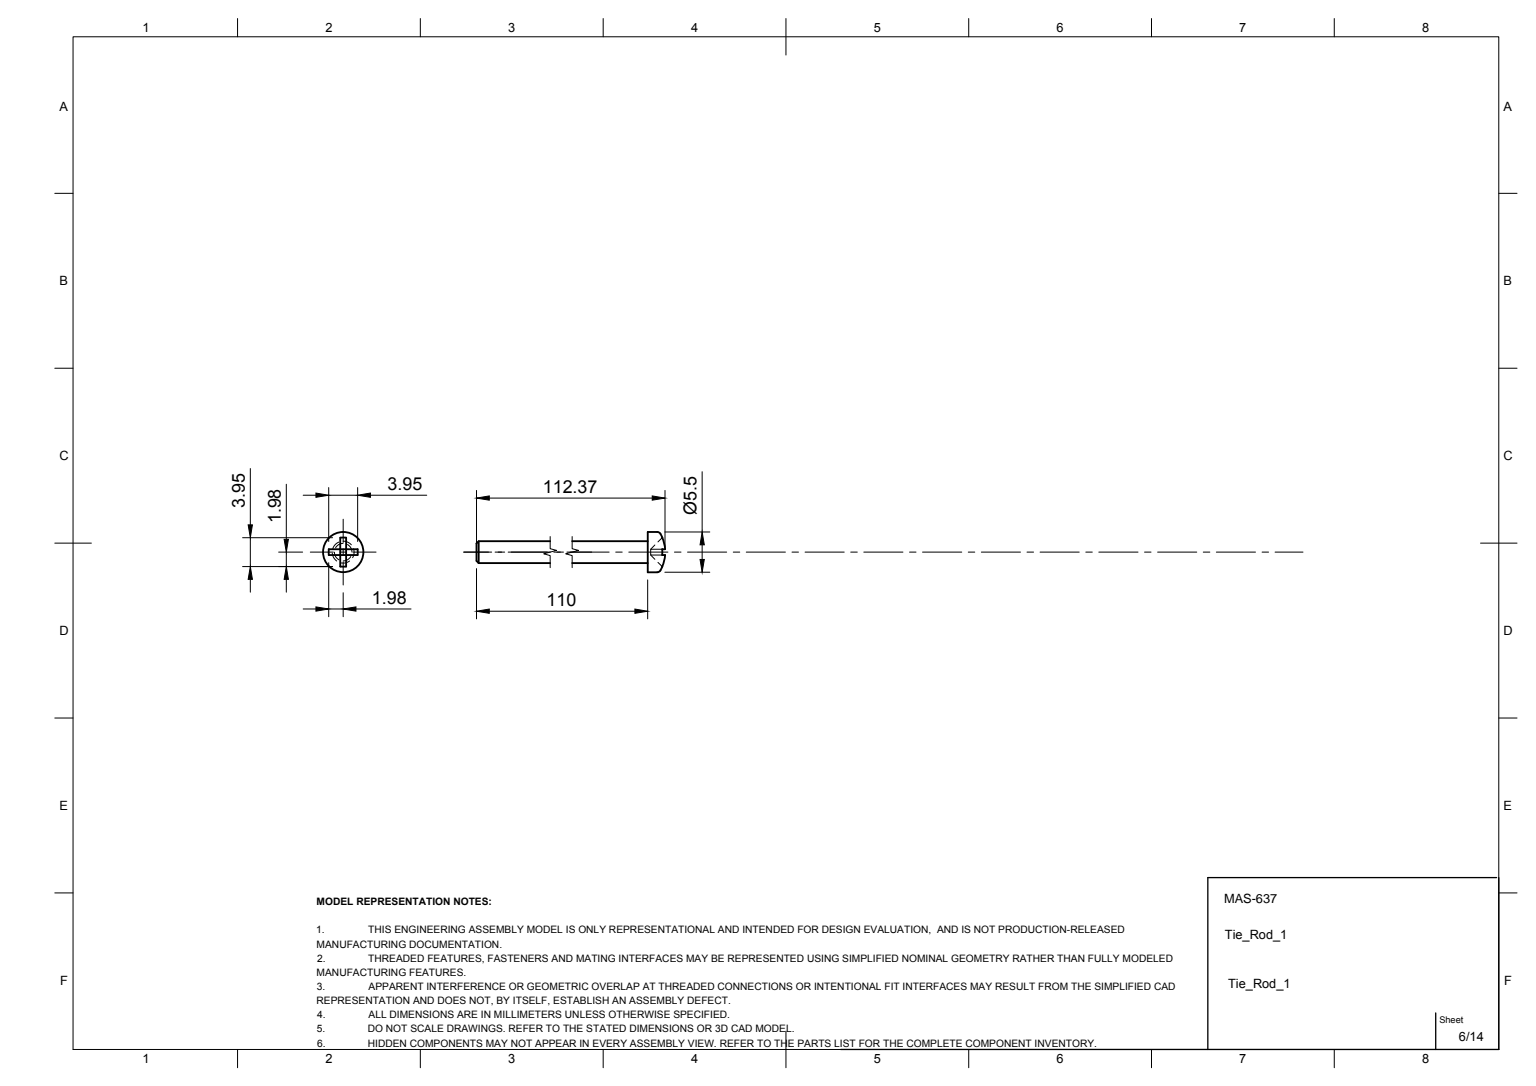
ISO-10303-21;
HEADER;
FILE_DESCRIPTION((''),'2;1');
FILE_NAME('Tie_Rod_1.step','2026-10-09T10:11:57-07:00',(''),(''),'','','');
FILE_SCHEMA (('AUTOMOTIVE_DESIGN { 1 0 10303 214 3 1 1 }'));
ENDSEC;
DATA;
#10=MECHANICAL_DESIGN_GEOMETRIC_PRESENTATION_REPRESENTATION('',(#126),#13510);
#71=SPHERICAL_SURFACE('',#8066,5.) ;
#96=SHAPE_REPRESENTATION_RELATIONSHIP('SRR','None',#13566,#111) ;
#111=ADVANCED_BREP_SHAPE_REPRESENTATION('',(#158),#13498) ;
#126=STYLED_ITEM('',(#13650),#158) ;
#158=MANIFOLD_SOLID_BREP('Body1',#7375) ;
#240=FACE_BOUND('',#1372,.T.) ;
#352=PLANE('',#8051) ;
#353=PLANE('',#8052) ;
#354=PLANE('',#8053) ;
#355=PLANE('',#8055) ;
#356=PLANE('',#8057) ;
#357=PLANE('',#8060) ;
#358=PLANE('',#8062) ;
#359=PLANE('',#8064) ;
#360=PLANE('',#8074) ;
#361=PLANE('',#8075) ;
#362=PLANE('',#8076) ;
#363=PLANE('',#8077) ;
#364=PLANE('',#8078) ;
#365=PLANE('',#8079) ;
#366=PLANE('',#8080) ;
#498=TOROIDAL_SURFACE('',#8040,2.25,0.5) ;
#632=CYLINDRICAL_SURFACE('',#8044,2.75) ;
#633=CYLINDRICAL_SURFACE('',#8046,1.5) ;
#866=FACE_OUTER_BOUND('',#1367,.T.) ;
#867=FACE_OUTER_BOUND('',#1368,.T.) ;
#868=FACE_OUTER_BOUND('',#1369,.T.) ;
#869=FACE_OUTER_BOUND('',#1370,.T.) ;
#870=FACE_OUTER_BOUND('',#1371,.T.) ;
#871=FACE_OUTER_BOUND('',#1373,.T.) ;
#872=FACE_OUTER_BOUND('',#1374,.T.) ;
#873=FACE_OUTER_BOUND('',#1375,.T.) ;
#874=FACE_OUTER_BOUND('',#1376,.T.) ;
#875=FACE_OUTER_BOUND('',#1377,.T.) ;
#876=FACE_OUTER_BOUND('',#1378,.T.) ;
#877=FACE_OUTER_BOUND('',#1379,.T.) ;
#878=FACE_OUTER_BOUND('',#1380,.T.) ;
#879=FACE_OUTER_BOUND('',#1381,.T.) ;
#880=FACE_OUTER_BOUND('',#1382,.T.) ;
#881=FACE_OUTER_BOUND('',#1383,.T.) ;
#882=FACE_OUTER_BOUND('',#1384,.T.) ;
#883=FACE_OUTER_BOUND('',#1385,.T.) ;
#884=FACE_OUTER_BOUND('',#1386,.T.) ;
#885=FACE_OUTER_BOUND('',#1387,.T.) ;
#1367=EDGE_LOOP('',(#5906,#5907,#5908,#5909)) ;
#1368=EDGE_LOOP('',(#5910,#5911,#5912,#5913)) ;
#1369=EDGE_LOOP('',(#5914,#5915,#5916,#5917)) ;
#1370=EDGE_LOOP('',(#5918,#5919,#5920,#5921)) ;
#1371=EDGE_LOOP('',(#5922)) ;
#1372=EDGE_LOOP('',(#5923)) ;
#1373=EDGE_LOOP('',(#5924)) ;
#1374=EDGE_LOOP('',(#5925,#5926,#5927,#5928)) ;
#1375=EDGE_LOOP('',(#5929,#5930,#5931,#5932)) ;
#1376=EDGE_LOOP('',(#5933,#5934,#5935,#5936)) ;
#1377=EDGE_LOOP('',(#5937,#5938,#5939)) ;
#1378=EDGE_LOOP('',(#5940,#5941,#5942)) ;
#1379=EDGE_LOOP('',(#5943,#5944,#5945)) ;
#1380=EDGE_LOOP('',(#5946,#5947,#5948,#5949,#5950,#5951,#5952,#5953,#5954,
#5955,#5956,#5957,#5958,#5959,#5960,#5961)) ;
#1381=EDGE_LOOP('',(#5962,#5963,#5964)) ;
#1382=EDGE_LOOP('',(#5965,#5966,#5967,#5968)) ;
#1383=EDGE_LOOP('',(#5969,#5970,#5971)) ;
#1384=EDGE_LOOP('',(#5972,#5973,#5974)) ;
#1385=EDGE_LOOP('',(#5975,#5976,#5977,#5978)) ;
#1386=EDGE_LOOP('',(#5979,#5980,#5981)) ;
#1387=EDGE_LOOP('',(#5982,#5983,#5984,#5985)) ;
#1906=LINE('',#12420,#2400) ;
#1907=LINE('',#12425,#2401) ;
#1908=LINE('',#12429,#2402) ;
#1909=LINE('',#12436,#2403) ;
#1910=LINE('',#12438,#2404) ;
#1911=LINE('',#12440,#2405) ;
#1912=LINE('',#12447,#2406) ;
#1913=LINE('',#12449,#2407) ;
#1914=LINE('',#12450,#2408) ;
#1915=LINE('',#12453,#2409) ;
#1916=LINE('',#12459,#2410) ;
#1917=LINE('',#12464,#2411) ;
#1918=LINE('',#12468,#2412) ;
#1919=LINE('',#12482,#2413) ;
#1920=LINE('',#12484,#2414) ;
#1921=LINE('',#12485,#2415) ;
#1922=LINE('',#12488,#2416) ;
#1923=LINE('',#12490,#2417) ;
#1924=LINE('',#12491,#2418) ;
#2400=VECTOR('',#9776,2.75) ;
#2401=VECTOR('',#9781,1.5) ;
#2402=VECTOR('',#9786,1.2) ;
#2403=VECTOR('',#9795,1.00000000000064) ;
#2404=VECTOR('',#9796,1.) ;
#2405=VECTOR('',#9797,1.00000000000064) ;
#2406=VECTOR('',#9804,1.00000000000064) ;
#2407=VECTOR('',#9805,1.) ;
#2408=VECTOR('',#9806,1.00000000000064) ;
#2409=VECTOR('',#9809,1.) ;
#2410=VECTOR('',#9816,1.) ;
#2411=VECTOR('',#9823,1.) ;
#2412=VECTOR('',#9828,1.) ;
#2413=VECTOR('',#9847,1.00000000000064) ;
#2414=VECTOR('',#9850,1.00000000000064) ;
#2415=VECTOR('',#9851,1.) ;
#2416=VECTOR('',#9856,1.00000000000064) ;
#2417=VECTOR('',#9859,1.) ;
#2418=VECTOR('',#9860,1.00000000000064) ;
#2898=CIRCLE('',#8041,2.75) ;
#2899=CIRCLE('',#8042,0.5) ;
#2900=CIRCLE('',#8043,2.5) ;
#2901=CIRCLE('',#8045,2.75) ;
#2902=CIRCLE('',#8047,1.5) ;
#2903=CIRCLE('',#8048,1.5) ;
#2904=CIRCLE('',#8050,1.2) ;
#2905=CIRCLE('',#8054,4.64997588898226) ;
#2906=CIRCLE('',#8056,4.64997588898056) ;
#2907=CIRCLE('',#8058,4.98397431775085) ;
#2908=CIRCLE('',#8059,4.98397431775085) ;
#2909=CIRCLE('',#8061,4.9839617983173) ;
#2910=CIRCLE('',#8063,4.98396179831711) ;
#2911=CIRCLE('',#8065,4.98397431775085) ;
#2912=CIRCLE('',#8067,5.) ;
#2913=CIRCLE('',#8068,4.98397431775085) ;
#2914=CIRCLE('',#8069,4.64973117502507) ;
#2915=CIRCLE('',#8070,4.98397431775085) ;
#2916=CIRCLE('',#8071,4.98397431775085) ;
#2917=CIRCLE('',#8072,4.64973117502507) ;
#2918=CIRCLE('',#8073,4.98397431775085) ;
#3496=VERTEX_POINT('',#12412) ;
#3497=VERTEX_POINT('',#12414) ;
#3498=VERTEX_POINT('',#12418) ;
#3499=VERTEX_POINT('',#12422) ;
#3500=VERTEX_POINT('',#12424) ;
#3501=VERTEX_POINT('',#12428) ;
#3502=VERTEX_POINT('',#12434) ;
#3503=VERTEX_POINT('',#12435) ;
#3504=VERTEX_POINT('',#12437) ;
#3505=VERTEX_POINT('',#12439) ;
#3506=VERTEX_POINT('',#12443) ;
#3507=VERTEX_POINT('',#12444) ;
#3508=VERTEX_POINT('',#12446) ;
#3509=VERTEX_POINT('',#12448) ;
#3510=VERTEX_POINT('',#12452) ;
#3511=VERTEX_POINT('',#12454) ;
#3512=VERTEX_POINT('',#12458) ;
#3513=VERTEX_POINT('',#12462) ;
#3514=VERTEX_POINT('',#12466) ;
#3515=VERTEX_POINT('',#12471) ;
#3516=VERTEX_POINT('',#12473) ;
#3517=VERTEX_POINT('',#12476) ;
#3518=VERTEX_POINT('',#12478) ;
#4340=EDGE_CURVE('',#3496,#3496,#2898,.T.) ;
#4341=EDGE_CURVE('',#3496,#3497,#2899,.T.) ;
#4342=EDGE_CURVE('',#3497,#3497,#2900,.T.) ;
#4343=EDGE_CURVE('',#3498,#3498,#2901,.T.) ;
#4344=EDGE_CURVE('',#3498,#3496,#1906,.T.) ;
#4345=EDGE_CURVE('',#3499,#3499,#2902,.T.) ;
#4346=EDGE_CURVE('',#3499,#3500,#1907,.T.) ;
#4347=EDGE_CURVE('',#3500,#3500,#2903,.T.) ;
#4348=EDGE_CURVE('',#3499,#3501,#1908,.T.) ;
#4349=EDGE_CURVE('',#3501,#3501,#2904,.F.) ;
#4350=EDGE_CURVE('',#3502,#3503,#1909,.T.) ;
#4351=EDGE_CURVE('',#3502,#3504,#1910,.F.) ;
#4352=EDGE_CURVE('',#3504,#3505,#1911,.T.) ;
#4353=EDGE_CURVE('',#3505,#3503,#2905,.T.) ;
#4354=EDGE_CURVE('',#3506,#3507,#2906,.T.) ;
#4355=EDGE_CURVE('',#3506,#3508,#1912,.F.) ;
#4356=EDGE_CURVE('',#3509,#3508,#1913,.F.) ;
#4357=EDGE_CURVE('',#3507,#3509,#1914,.F.) ;
#4358=EDGE_CURVE('',#3504,#3510,#1915,.T.) ;
#4359=EDGE_CURVE('',#3511,#3510,#2907,.F.) ;
#4360=EDGE_CURVE('',#3505,#3511,#2908,.F.) ;
#4361=EDGE_CURVE('',#3508,#3512,#1916,.T.) ;
#4362=EDGE_CURVE('',#3512,#3506,#2909,.T.) ;
#4363=EDGE_CURVE('',#3513,#3503,#2910,.T.) ;
#4364=EDGE_CURVE('',#3502,#3513,#1917,.T.) ;
#4365=EDGE_CURVE('',#3507,#3514,#2911,.F.) ;
#4366=EDGE_CURVE('',#3509,#3514,#1918,.T.) ;
#4367=EDGE_CURVE('',#3497,#3511,#2912,.T.) ;
#4368=EDGE_CURVE('',#3515,#3510,#2913,.T.) ;
#4369=EDGE_CURVE('',#3516,#3515,#2914,.T.) ;
#4370=EDGE_CURVE('',#3516,#3512,#2915,.T.) ;
#4371=EDGE_CURVE('',#3517,#3514,#2916,.T.) ;
#4372=EDGE_CURVE('',#3517,#3518,#2917,.T.) ;
#4373=EDGE_CURVE('',#3518,#3513,#2918,.T.) ;
#4374=EDGE_CURVE('',#3518,#3502,#1919,.F.) ;
#4375=EDGE_CURVE('',#3517,#3509,#1920,.F.) ;
#4376=EDGE_CURVE('',#3509,#3502,#1921,.T.) ;
#4377=EDGE_CURVE('',#3504,#3515,#1922,.T.) ;
#4378=EDGE_CURVE('',#3508,#3504,#1923,.T.) ;
#4379=EDGE_CURVE('',#3508,#3516,#1924,.T.) ;
#5906=ORIENTED_EDGE('',*,*,#4340,.F.) ;
#5907=ORIENTED_EDGE('',*,*,#4341,.T.) ;
#5908=ORIENTED_EDGE('',*,*,#4342,.T.) ;
#5909=ORIENTED_EDGE('',*,*,#4341,.F.) ;
#5910=ORIENTED_EDGE('',*,*,#4343,.F.) ;
#5911=ORIENTED_EDGE('',*,*,#4344,.T.) ;
#5912=ORIENTED_EDGE('',*,*,#4340,.T.) ;
#5913=ORIENTED_EDGE('',*,*,#4344,.F.) ;
#5914=ORIENTED_EDGE('',*,*,#4345,.F.) ;
#5915=ORIENTED_EDGE('',*,*,#4346,.T.) ;
#5916=ORIENTED_EDGE('',*,*,#4347,.T.) ;
#5917=ORIENTED_EDGE('',*,*,#4346,.F.) ;
#5918=ORIENTED_EDGE('',*,*,#4345,.T.) ;
#5919=ORIENTED_EDGE('',*,*,#4348,.T.) ;
#5920=ORIENTED_EDGE('',*,*,#4349,.F.) ;
#5921=ORIENTED_EDGE('',*,*,#4348,.F.) ;
#5922=ORIENTED_EDGE('',*,*,#4343,.T.) ;
#5923=ORIENTED_EDGE('',*,*,#4347,.F.) ;
#5924=ORIENTED_EDGE('',*,*,#4349,.T.) ;
#5925=ORIENTED_EDGE('',*,*,#4350,.F.) ;
#5926=ORIENTED_EDGE('',*,*,#4351,.T.) ;
#5927=ORIENTED_EDGE('',*,*,#4352,.T.) ;
#5928=ORIENTED_EDGE('',*,*,#4353,.T.) ;
#5929=ORIENTED_EDGE('',*,*,#4354,.F.) ;
#5930=ORIENTED_EDGE('',*,*,#4355,.T.) ;
#5931=ORIENTED_EDGE('',*,*,#4356,.F.) ;
#5932=ORIENTED_EDGE('',*,*,#4357,.F.) ;
#5933=ORIENTED_EDGE('',*,*,#4358,.T.) ;
#5934=ORIENTED_EDGE('',*,*,#4359,.F.) ;
#5935=ORIENTED_EDGE('',*,*,#4360,.F.) ;
#5936=ORIENTED_EDGE('',*,*,#4352,.F.) ;
#5937=ORIENTED_EDGE('',*,*,#4361,.F.) ;
#5938=ORIENTED_EDGE('',*,*,#4355,.F.) ;
#5939=ORIENTED_EDGE('',*,*,#4362,.F.) ;
#5940=ORIENTED_EDGE('',*,*,#4350,.T.) ;
#5941=ORIENTED_EDGE('',*,*,#4363,.F.) ;
#5942=ORIENTED_EDGE('',*,*,#4364,.F.) ;
#5943=ORIENTED_EDGE('',*,*,#4365,.F.) ;
#5944=ORIENTED_EDGE('',*,*,#4357,.T.) ;
#5945=ORIENTED_EDGE('',*,*,#4366,.T.) ;
#5946=ORIENTED_EDGE('',*,*,#4342,.F.) ;
#5947=ORIENTED_EDGE('',*,*,#4367,.T.) ;
#5948=ORIENTED_EDGE('',*,*,#4359,.T.) ;
#5949=ORIENTED_EDGE('',*,*,#4368,.F.) ;
#5950=ORIENTED_EDGE('',*,*,#4369,.F.) ;
#5951=ORIENTED_EDGE('',*,*,#4370,.T.) ;
#5952=ORIENTED_EDGE('',*,*,#4362,.T.) ;
#5953=ORIENTED_EDGE('',*,*,#4354,.T.) ;
#5954=ORIENTED_EDGE('',*,*,#4365,.T.) ;
#5955=ORIENTED_EDGE('',*,*,#4371,.F.) ;
#5956=ORIENTED_EDGE('',*,*,#4372,.T.) ;
#5957=ORIENTED_EDGE('',*,*,#4373,.T.) ;
#5958=ORIENTED_EDGE('',*,*,#4363,.T.) ;
#5959=ORIENTED_EDGE('',*,*,#4353,.F.) ;
#5960=ORIENTED_EDGE('',*,*,#4360,.T.) ;
#5961=ORIENTED_EDGE('',*,*,#4367,.F.) ;
#5962=ORIENTED_EDGE('',*,*,#4374,.T.) ;
#5963=ORIENTED_EDGE('',*,*,#4364,.T.) ;
#5964=ORIENTED_EDGE('',*,*,#4373,.F.) ;
#5965=ORIENTED_EDGE('',*,*,#4374,.F.) ;
#5966=ORIENTED_EDGE('',*,*,#4372,.F.) ;
#5967=ORIENTED_EDGE('',*,*,#4375,.T.) ;
#5968=ORIENTED_EDGE('',*,*,#4376,.T.) ;
#5969=ORIENTED_EDGE('',*,*,#4371,.T.) ;
#5970=ORIENTED_EDGE('',*,*,#4366,.F.) ;
#5971=ORIENTED_EDGE('',*,*,#4375,.F.) ;
#5972=ORIENTED_EDGE('',*,*,#4377,.T.) ;
#5973=ORIENTED_EDGE('',*,*,#4368,.T.) ;
#5974=ORIENTED_EDGE('',*,*,#4358,.F.) ;
#5975=ORIENTED_EDGE('',*,*,#4377,.F.) ;
#5976=ORIENTED_EDGE('',*,*,#4378,.F.) ;
#5977=ORIENTED_EDGE('',*,*,#4379,.T.) ;
#5978=ORIENTED_EDGE('',*,*,#4369,.T.) ;
#5979=ORIENTED_EDGE('',*,*,#4361,.T.) ;
#5980=ORIENTED_EDGE('',*,*,#4370,.F.) ;
#5981=ORIENTED_EDGE('',*,*,#4379,.F.) ;
#5982=ORIENTED_EDGE('',*,*,#4378,.T.) ;
#5983=ORIENTED_EDGE('',*,*,#4351,.F.) ;
#5984=ORIENTED_EDGE('',*,*,#4376,.F.) ;
#5985=ORIENTED_EDGE('',*,*,#4356,.T.) ;
#6885=CONICAL_SURFACE('',#8049,1.2,0.785398163397) ;
#7116=ADVANCED_FACE('',(#866),#498,.T.) ;
#7117=ADVANCED_FACE('',(#867),#632,.T.) ;
#7118=ADVANCED_FACE('',(#868),#633,.T.) ;
#7119=ADVANCED_FACE('',(#869),#6885,.T.) ;
#7120=ADVANCED_FACE('',(#870,#240),#352,.T.) ;
#7121=ADVANCED_FACE('',(#871),#353,.T.) ;
#7122=ADVANCED_FACE('',(#872),#354,.T.) ;
#7123=ADVANCED_FACE('',(#873),#355,.F.) ;
#7124=ADVANCED_FACE('',(#874),#356,.F.) ;
#7125=ADVANCED_FACE('',(#875),#357,.F.) ;
#7126=ADVANCED_FACE('',(#876),#358,.T.) ;
#7127=ADVANCED_FACE('',(#877),#359,.T.) ;
#7128=ADVANCED_FACE('',(#878),#71,.T.) ;
#7129=ADVANCED_FACE('',(#879),#360,.T.) ;
#7130=ADVANCED_FACE('',(#880),#361,.F.) ;
#7131=ADVANCED_FACE('',(#881),#362,.F.) ;
#7132=ADVANCED_FACE('',(#882),#363,.T.) ;
#7133=ADVANCED_FACE('',(#883),#364,.T.) ;
#7134=ADVANCED_FACE('',(#884),#365,.F.) ;
#7135=ADVANCED_FACE('',(#885),#366,.F.) ;
#7375=CLOSED_SHELL('',(#7116,#7117,#7118,#7119,#7120,#7121,#7122,#7123,
#7124,#7125,#7126,#7127,#7128,#7129,#7130,#7131,#7132,#7133,#7134,#7135)) ;
#8039=AXIS2_PLACEMENT_3D('',#12410,#9762,#9763) ;
#8040=AXIS2_PLACEMENT_3D('',#12411,#9764,#9765) ;
#8041=AXIS2_PLACEMENT_3D('',#12413,#9766,#9767) ;
#8042=AXIS2_PLACEMENT_3D('',#12415,#9768,#9769) ;
#8043=AXIS2_PLACEMENT_3D('',#12416,#9770,#9771) ;
#8044=AXIS2_PLACEMENT_3D('',#12417,#9772,#9773) ;
#8045=AXIS2_PLACEMENT_3D('',#12419,#9774,#9775) ;
#8046=AXIS2_PLACEMENT_3D('',#12421,#9777,#9778) ;
#8047=AXIS2_PLACEMENT_3D('',#12423,#9779,#9780) ;
#8048=AXIS2_PLACEMENT_3D('',#12426,#9782,#9783) ;
#8049=AXIS2_PLACEMENT_3D('',#12427,#9784,#9785) ;
#8050=AXIS2_PLACEMENT_3D('',#12430,#9787,#9788) ;
#8051=AXIS2_PLACEMENT_3D('',#12431,#9789,#9790) ;
#8052=AXIS2_PLACEMENT_3D('',#12432,#9791,#9792) ;
#8053=AXIS2_PLACEMENT_3D('',#12433,#9793,#9794) ;
#8054=AXIS2_PLACEMENT_3D('',#12441,#9798,#9799) ;
#8055=AXIS2_PLACEMENT_3D('',#12442,#9800,#9801) ;
#8056=AXIS2_PLACEMENT_3D('',#12445,#9802,#9803) ;
#8057=AXIS2_PLACEMENT_3D('',#12451,#9807,#9808) ;
#8058=AXIS2_PLACEMENT_3D('',#12455,#9810,#9811) ;
#8059=AXIS2_PLACEMENT_3D('',#12456,#9812,#9813) ;
#8060=AXIS2_PLACEMENT_3D('',#12457,#9814,#9815) ;
#8061=AXIS2_PLACEMENT_3D('',#12460,#9817,#9818) ;
#8062=AXIS2_PLACEMENT_3D('',#12461,#9819,#9820) ;
#8063=AXIS2_PLACEMENT_3D('',#12463,#9821,#9822) ;
#8064=AXIS2_PLACEMENT_3D('',#12465,#9824,#9825) ;
#8065=AXIS2_PLACEMENT_3D('',#12467,#9826,#9827) ;
#8066=AXIS2_PLACEMENT_3D('',#12469,#9829,#9830) ;
#8067=AXIS2_PLACEMENT_3D('',#12470,#9831,#9832) ;
#8068=AXIS2_PLACEMENT_3D('',#12472,#9833,#9834) ;
#8069=AXIS2_PLACEMENT_3D('',#12474,#9835,#9836) ;
#8070=AXIS2_PLACEMENT_3D('',#12475,#9837,#9838) ;
#8071=AXIS2_PLACEMENT_3D('',#12477,#9839,#9840) ;
#8072=AXIS2_PLACEMENT_3D('',#12479,#9841,#9842) ;
#8073=AXIS2_PLACEMENT_3D('',#12480,#9843,#9844) ;
#8074=AXIS2_PLACEMENT_3D('',#12481,#9845,#9846) ;
#8075=AXIS2_PLACEMENT_3D('',#12483,#9848,#9849) ;
#8076=AXIS2_PLACEMENT_3D('',#12486,#9852,#9853) ;
#8077=AXIS2_PLACEMENT_3D('',#12487,#9854,#9855) ;
#8078=AXIS2_PLACEMENT_3D('',#12489,#9857,#9858) ;
#8079=AXIS2_PLACEMENT_3D('',#12492,#9861,#9862) ;
#8080=AXIS2_PLACEMENT_3D('',#12493,#9863,#9864) ;
#9762=DIRECTION('axis',(0.,0.,1.)) ;
#9763=DIRECTION('refdir',(1.,0.,0.)) ;
#9764=DIRECTION('center_axis',(0.,0.,1.)) ;
#9765=DIRECTION('ref_axis',(-0.479425538604204,0.877582561890372,0.)) ;
#9766=DIRECTION('center_axis',(0.,0.,1.)) ;
#9767=DIRECTION('ref_axis',(-1.,0.,0.)) ;
#9768=DIRECTION('center_axis',(0.877582561890372,0.479425538604204,0.)) ;
#9769=DIRECTION('ref_axis',(0.479425538604204,-0.877582561890372,0.)) ;
#9770=DIRECTION('center_axis',(0.,0.,1.)) ;
#9771=DIRECTION('ref_axis',(-1.,0.,0.)) ;
#9772=DIRECTION('center_axis',(0.,0.,1.)) ;
#9773=DIRECTION('ref_axis',(-0.479425538604204,0.877582561890372,0.)) ;
#9774=DIRECTION('center_axis',(0.,0.,1.)) ;
#9775=DIRECTION('ref_axis',(-1.,0.,0.)) ;
#9776=DIRECTION('',(0.,0.,-1.)) ;
#9777=DIRECTION('center_axis',(0.,0.,1.)) ;
#9778=DIRECTION('ref_axis',(-0.479425538604204,0.877582561890372,0.)) ;
#9779=DIRECTION('center_axis',(0.,0.,1.)) ;
#9780=DIRECTION('ref_axis',(-1.,0.,0.)) ;
#9781=DIRECTION('',(0.,0.,-1.)) ;
#9782=DIRECTION('center_axis',(0.,0.,1.)) ;
#9783=DIRECTION('ref_axis',(-1.,0.,0.)) ;
#9784=DIRECTION('center_axis',(0.,0.,-1.)) ;
#9785=DIRECTION('ref_axis',(-0.479425538604203,0.877582561890373,0.)) ;
#9786=DIRECTION('',(-0.339005049420893,0.620544580563467,0.707106781186865)) ;
#9787=DIRECTION('center_axis',(0.,0.,-1.)) ;
#9788=DIRECTION('ref_axis',(1.,0.,0.)) ;
#9789=DIRECTION('center_axis',(0.,0.,1.)) ;
#9790=DIRECTION('ref_axis',(1.,0.,0.)) ;
#9791=DIRECTION('center_axis',(0.,0.,1.)) ;
#9792=DIRECTION('ref_axis',(1.,0.,0.)) ;
#9793=DIRECTION('center_axis',(0.,0.707106781186548,-0.707106781186548)) ;
#9794=DIRECTION('ref_axis',(0.,-0.707106781186548,-0.707106781186548)) ;
#9795=DIRECTION('',(0.,-0.707106781186548,-0.707106781186548)) ;
#9796=DIRECTION('',(-1.,0.,0.)) ;
#9797=DIRECTION('',(0.,-0.707106781186548,-0.707106781186548)) ;
#9798=DIRECTION('center_axis',(0.,0.70710678018955,-0.707106782183545)) ;
#9799=DIRECTION('ref_axis',(-0.0860219514143675,-0.704485708397953,-0.70448570641135)) ;
#9800=DIRECTION('center_axis',(0.,0.707106781186548,0.707106781186548)) ;
#9801=DIRECTION('ref_axis',(0.,0.707106781186548,-0.707106781186548)) ;
#9802=DIRECTION('center_axis',(0.,0.707106780189292,0.707106782183803)) ;
#9803=DIRECTION('ref_axis',(-0.0860219514143926,0.704485708398209,-0.704485706411091)) ;
#9804=DIRECTION('',(0.,0.707106781186548,-0.707106781186548)) ;
#9805=DIRECTION('',(-1.,0.,0.)) ;
#9806=DIRECTION('',(0.,0.707106781186548,-0.707106781186548)) ;
#9807=DIRECTION('center_axis',(1.,0.,0.)) ;
#9808=DIRECTION('ref_axis',(0.,1.,0.)) ;
#9809=DIRECTION('',(0.,0.,-1.)) ;
#9810=DIRECTION('center_axis',(-1.,0.,0.)) ;
#9811=DIRECTION('ref_axis',(0.,0.,1.)) ;
#9812=DIRECTION('center_axis',(-1.,0.,0.)) ;
#9813=DIRECTION('ref_axis',(0.,0.,1.)) ;
#9814=DIRECTION('center_axis',(1.,0.,0.)) ;
#9815=DIRECTION('ref_axis',(0.,1.,0.)) ;
#9816=DIRECTION('',(0.,0.,-1.)) ;
#9817=DIRECTION('center_axis',(1.,0.,0.)) ;
#9818=DIRECTION('ref_axis',(0.,0.396404687454843,-0.918075881266809)) ;
#9819=DIRECTION('center_axis',(1.,0.,0.)) ;
#9820=DIRECTION('ref_axis',(0.,1.,0.)) ;
#9821=DIRECTION('center_axis',(-1.,0.,0.)) ;
#9822=DIRECTION('ref_axis',(0.,-0.396404687454847,-0.918075881266807)) ;
#9823=DIRECTION('',(0.,0.,-1.)) ;
#9824=DIRECTION('center_axis',(1.,0.,0.)) ;
#9825=DIRECTION('ref_axis',(0.,1.,0.)) ;
#9826=DIRECTION('center_axis',(1.,0.,0.)) ;
#9827=DIRECTION('ref_axis',(0.,0.,1.)) ;
#9828=DIRECTION('',(0.,0.,-1.)) ;
#9829=DIRECTION('center_axis',(-8.80690426921701E-17,0.,1.)) ;
#9830=DIRECTION('ref_axis',(-0.479425538604204,0.877582561890372,0.)) ;
#9831=DIRECTION('center_axis',(0.877582561890372,0.479425538604204,5.15252374060181E-17)) ;
#9832=DIRECTION('ref_axis',(0.479425538604204,-0.877582561890372,0.)) ;
#9833=DIRECTION('center_axis',(6.12323399574E-17,1.,0.)) ;
#9834=DIRECTION('ref_axis',(0.,0.,-1.)) ;
#9835=DIRECTION('center_axis',(-0.707106781186548,4.32978028117723E-17,
-0.707106781186548)) ;
#9836=DIRECTION('ref_axis',(2.73536852476314E-32,-1.,-6.12323399573643E-17)) ;
#9837=DIRECTION('center_axis',(6.12323399574E-17,1.,0.)) ;
#9838=DIRECTION('ref_axis',(0.,0.,-1.)) ;
#9839=DIRECTION('center_axis',(-6.12323399574E-17,-1.,0.)) ;
#9840=DIRECTION('ref_axis',(0.,0.,-1.)) ;
#9841=DIRECTION('center_axis',(-0.707106781186548,4.32978028117723E-17,
0.707106781186548)) ;
#9842=DIRECTION('ref_axis',(-2.73536852476314E-32,1.,-6.12323399573643E-17)) ;
#9843=DIRECTION('center_axis',(-6.12323399574E-17,-1.,0.)) ;
#9844=DIRECTION('ref_axis',(0.,0.,-1.)) ;
#9845=DIRECTION('center_axis',(6.12323399574E-17,1.,0.)) ;
#9846=DIRECTION('ref_axis',(-1.,6.12323399574E-17,0.)) ;
#9847=DIRECTION('',(-0.707106781186548,0.,-0.707106781186548)) ;
#9848=DIRECTION('center_axis',(-0.707106781186548,4.32978028117723E-17,
0.707106781186548)) ;
#9849=DIRECTION('ref_axis',(-0.707106781186548,4.32978028117723E-17,-0.707106781186548)) ;
#9850=DIRECTION('',(-0.707106781186548,0.,-0.707106781186548)) ;
#9851=DIRECTION('',(0.,-1.,0.)) ;
#9852=DIRECTION('center_axis',(6.12323399574E-17,1.,0.)) ;
#9853=DIRECTION('ref_axis',(-1.,6.12323399574E-17,0.)) ;
#9854=DIRECTION('center_axis',(6.12323399574E-17,1.,0.)) ;
#9855=DIRECTION('ref_axis',(-1.,6.12323399574E-17,0.)) ;
#9856=DIRECTION('',(0.707106781186548,0.,-0.707106781186548)) ;
#9857=DIRECTION('center_axis',(-0.707106781186548,4.32978028117723E-17,
-0.707106781186548)) ;
#9858=DIRECTION('ref_axis',(0.707106781186548,-4.32978028117723E-17,-0.707106781186548)) ;
#9859=DIRECTION('',(0.,-1.,0.)) ;
#9860=DIRECTION('',(0.707106781186548,0.,-0.707106781186548)) ;
#9861=DIRECTION('center_axis',(6.12323399574E-17,1.,0.)) ;
#9862=DIRECTION('ref_axis',(-1.,6.12323399574E-17,0.)) ;
#9863=DIRECTION('center_axis',(0.,0.,1.)) ;
#9864=DIRECTION('ref_axis',(0.,1.,0.)) ;
#12410=CARTESIAN_POINT('',(0.,0.,0.)) ;
#12411=CARTESIAN_POINT('Origin',(0.,25.,7.50288568297)) ;
#12412=CARTESIAN_POINT('',(1.31842023116156,22.5866479548015,7.50288568297)) ;
#12413=CARTESIAN_POINT('Origin',(0.,25.,7.50288568297)) ;
#12414=CARTESIAN_POINT('',(1.19856384651051,22.8060435952741,7.06987298108)) ;
#12415=CARTESIAN_POINT('Origin',(1.07870746185946,23.0254392357467,7.50288568297)) ;
#12416=CARTESIAN_POINT('Origin',(0.,25.,7.06987298108)) ;
#12417=CARTESIAN_POINT('Origin',(0.,25.,62.6)) ;
#12418=CARTESIAN_POINT('',(1.31842023116156,22.5866479548015,8.8)) ;
#12419=CARTESIAN_POINT('Origin',(0.,25.,8.8)) ;
#12420=CARTESIAN_POINT('',(1.31842023116156,22.5866479548015,62.6)) ;
#12421=CARTESIAN_POINT('Origin',(0.,25.,62.6)) ;
#12422=CARTESIAN_POINT('',(0.719138307906305,23.6836261571644,118.5)) ;
#12423=CARTESIAN_POINT('Origin',(0.,25.,118.5)) ;
#12424=CARTESIAN_POINT('',(0.719138307906305,23.6836261571644,8.8)) ;
#12425=CARTESIAN_POINT('',(0.719138307906306,23.6836261571644,62.6)) ;
#12426=CARTESIAN_POINT('Origin',(0.,25.,8.8)) ;
#12427=CARTESIAN_POINT('Origin',(0.,25.,118.8)) ;
#12428=CARTESIAN_POINT('',(0.575310646325044,23.9469009257316,118.8)) ;
#12429=CARTESIAN_POINT('',(0.575310646325043,23.9469009257316,118.8)) ;
#12430=CARTESIAN_POINT('Origin',(0.,25.,118.8)) ;
#12431=CARTESIAN_POINT('Origin',(0.,26.5,8.8)) ;
#12432=CARTESIAN_POINT('Origin',(0.,25.,118.8)) ;
#12433=CARTESIAN_POINT('Origin',(0.,24.6,8.4)) ;
#12434=CARTESIAN_POINT('',(-0.4,24.6,8.4)) ;
#12435=CARTESIAN_POINT('',(-0.400000008727488,23.024332247423,6.82433230687695)) ;
#12436=CARTESIAN_POINT('',(-0.4,23.8121660646,7.61216606458)) ;
#12437=CARTESIAN_POINT('',(0.4,24.6,8.4)) ;
#12438=CARTESIAN_POINT('',(-0.2,24.6,8.4)) ;
#12439=CARTESIAN_POINT('',(0.4,23.0243321292,6.82433212917)) ;
#12440=CARTESIAN_POINT('',(0.4,23.8121660646,7.61216606458)) ;
#12441=CARTESIAN_POINT('Origin',(1.19348975147204E-14,26.3001736873831,
10.1001736781154)) ;
#12442=CARTESIAN_POINT('Origin',(0.,25.4,8.4)) ;
#12443=CARTESIAN_POINT('',(0.400000008727487,26.975667752577,6.82433230687695)) ;
#12444=CARTESIAN_POINT('',(-0.4,26.9756678708,6.82433212917)) ;
#12445=CARTESIAN_POINT('Origin',(-1.67921232474555E-14,23.6998263126169,
10.100173678113)) ;
#12446=CARTESIAN_POINT('',(0.4,25.4,8.4)) ;
#12447=CARTESIAN_POINT('',(0.4,26.1878339354,7.61216606458)) ;
#12448=CARTESIAN_POINT('',(-0.4,25.4,8.4)) ;
#12449=CARTESIAN_POINT('',(0.2,25.4,8.4)) ;
#12450=CARTESIAN_POINT('',(-0.4,26.1878339354,7.61216606458)) ;
#12451=CARTESIAN_POINT('Origin',(0.4,0.,0.)) ;
#12452=CARTESIAN_POINT('',(0.40000000027355,24.5999999997533,6.43210306118567)) ;
#12453=CARTESIAN_POINT('',(0.4,24.6,7.41605197605)) ;
#12454=CARTESIAN_POINT('',(0.4,24.267804911315,6.47010239943002)) ;
#12455=CARTESIAN_POINT('Origin',(0.4,25.,11.4)) ;
#12456=CARTESIAN_POINT('Origin',(0.4,25.,11.4)) ;
#12457=CARTESIAN_POINT('Origin',(0.4,0.,0.)) ;
#12458=CARTESIAN_POINT('',(0.400000000037177,25.4000000002017,6.43210306142872)) ;
#12459=CARTESIAN_POINT('',(0.4,25.4,7.41605153106)) ;
#12460=CARTESIAN_POINT('Origin',(0.4,25.0000017211512,11.3999875801003)) ;
#12461=CARTESIAN_POINT('Origin',(-0.4,0.,0.)) ;
#12462=CARTESIAN_POINT('',(-0.400000000037177,24.5999999997983,6.43210306142873)) ;
#12463=CARTESIAN_POINT('Origin',(-0.4,24.9999982788488,11.3999875801001)) ;
#12464=CARTESIAN_POINT('',(-0.4,24.6,7.41605153106)) ;
#12465=CARTESIAN_POINT('Origin',(-0.4,0.,0.)) ;
#12466=CARTESIAN_POINT('',(-0.40000000027355,25.4000000002467,6.43210306118567)) ;
#12467=CARTESIAN_POINT('Origin',(-0.4,25.,11.4)) ;
#12468=CARTESIAN_POINT('',(-0.4,25.4,7.41605197605)) ;
#12469=CARTESIAN_POINT('Origin',(0.,25.,11.4)) ;
#12470=CARTESIAN_POINT('Origin',(0.,25.,11.4)) ;
#12471=CARTESIAN_POINT('',(1.97566787083,24.6,6.82433212917)) ;
#12472=CARTESIAN_POINT('Origin',(-2.44929359829597E-17,24.6,11.4)) ;
#12473=CARTESIAN_POINT('',(1.97566787029766,25.400000000087,6.82433212927802)) ;
#12474=CARTESIAN_POINT('Origin',(-1.3,25.,10.1)) ;
#12475=CARTESIAN_POINT('Origin',(2.44929359829601E-17,25.4,11.4)) ;
#12476=CARTESIAN_POINT('',(-1.97566787029766,25.400000000087,6.82433212927802)) ;
#12477=CARTESIAN_POINT('Origin',(2.44929359829601E-17,25.4,11.4)) ;
#12478=CARTESIAN_POINT('',(-1.97566787083,24.6,6.82433212917)) ;
#12479=CARTESIAN_POINT('Origin',(1.3,25.,10.1)) ;
#12480=CARTESIAN_POINT('Origin',(-2.44929359829597E-17,24.6,11.4)) ;
#12481=CARTESIAN_POINT('Origin',(25.,24.6,0.)) ;
#12482=CARTESIAN_POINT('',(-1.18783393542,24.6,7.61216606458)) ;
#12483=CARTESIAN_POINT('Origin',(-0.4,25.,8.4)) ;
#12484=CARTESIAN_POINT('',(-1.18783380997,25.4,7.61216619003)) ;
#12485=CARTESIAN_POINT('',(-0.4,25.2,8.4)) ;
#12486=CARTESIAN_POINT('Origin',(25.,25.4,0.)) ;
#12487=CARTESIAN_POINT('Origin',(25.,24.6,0.)) ;
#12488=CARTESIAN_POINT('',(1.18783393542,24.6,7.61216606458)) ;
#12489=CARTESIAN_POINT('Origin',(0.4,25.,8.4)) ;
#12490=CARTESIAN_POINT('',(0.4,24.8,8.4)) ;
#12491=CARTESIAN_POINT('',(1.18783380997,25.4,7.61216619003)) ;
#12492=CARTESIAN_POINT('Origin',(25.,25.4,0.)) ;
#12493=CARTESIAN_POINT('Origin',(0.,24.6,8.4)) ;
#13481=UNCERTAINTY_MEASURE_WITH_UNIT(LENGTH_MEASURE(0.01),#13511,
'DISTANCE_ACCURACY_VALUE',
'Maximum model space distance between geometric entities at asserted c
onnectivities') ;
#13493=UNCERTAINTY_MEASURE_WITH_UNIT(LENGTH_MEASURE(0.01),#13511,
'DISTANCE_ACCURACY_VALUE',
'Maximum model space distance between geometric entities at asserted c
onnectivities') ;
#13498=(
GEOMETRIC_REPRESENTATION_CONTEXT(3)
GLOBAL_UNCERTAINTY_ASSIGNED_CONTEXT((#13481))
GLOBAL_UNIT_ASSIGNED_CONTEXT((#13511,#13513,#13514))
REPRESENTATION_CONTEXT('','3D')
) ;
#13510=(
GEOMETRIC_REPRESENTATION_CONTEXT(3)
GLOBAL_UNCERTAINTY_ASSIGNED_CONTEXT((#13493))
GLOBAL_UNIT_ASSIGNED_CONTEXT((#13511,#13513,#13514))
REPRESENTATION_CONTEXT('','3D')
) ;
#13511=(
LENGTH_UNIT()
NAMED_UNIT(*)
SI_UNIT(.MILLI.,.METRE.)
) ;
#13513=(
NAMED_UNIT(*)
PLANE_ANGLE_UNIT()
SI_UNIT($,.RADIAN.)
) ;
#13514=(
NAMED_UNIT(*)
SI_UNIT($,.STERADIAN.)
SOLID_ANGLE_UNIT()
) ;
#13519=SHAPE_DEFINITION_REPRESENTATION(#13535,#13566) ;
#13535=PRODUCT_DEFINITION_SHAPE('',$,#13583) ;
#13566=SHAPE_REPRESENTATION('',(#8039),#13498) ;
#13578=PRODUCT_DEFINITION_CONTEXT('part definition',#13628,'design') ;
#13583=PRODUCT_DEFINITION('Tie_Rod_1','Tie_Rod_1',#13599,#13578) ;
#13599=PRODUCT_DEFINITION_FORMATION('',$,#13634) ;
#13628=APPLICATION_CONTEXT(
'Core Data for Automotive Mechanical Design Process') ;
#13629=PRODUCT_CONTEXT('part definition',#13628,'mechanical') ;
#13634=PRODUCT('Tie_Rod_1','Tie_Rod_1',$,(#13629)) ;
#13650=PRESENTATION_STYLE_ASSIGNMENT((#13655)) ;
#13655=SURFACE_STYLE_USAGE(.BOTH.,#13660) ;
#13660=SURFACE_SIDE_STYLE('',(#13665)) ;
#13665=SURFACE_STYLE_FILL_AREA(#13670) ;
#13670=FILL_AREA_STYLE('Opaque(144,144,144)',(#13675)) ;
#13675=FILL_AREA_STYLE_COLOUR('Opaque(144,144,144)',#13680) ;
#13680=COLOUR_RGB('Opaque(144,144,144)', 0.40784314, 0.44705882, 0.49803922) ;
ENDSEC;
END-ISO-10303-21;
